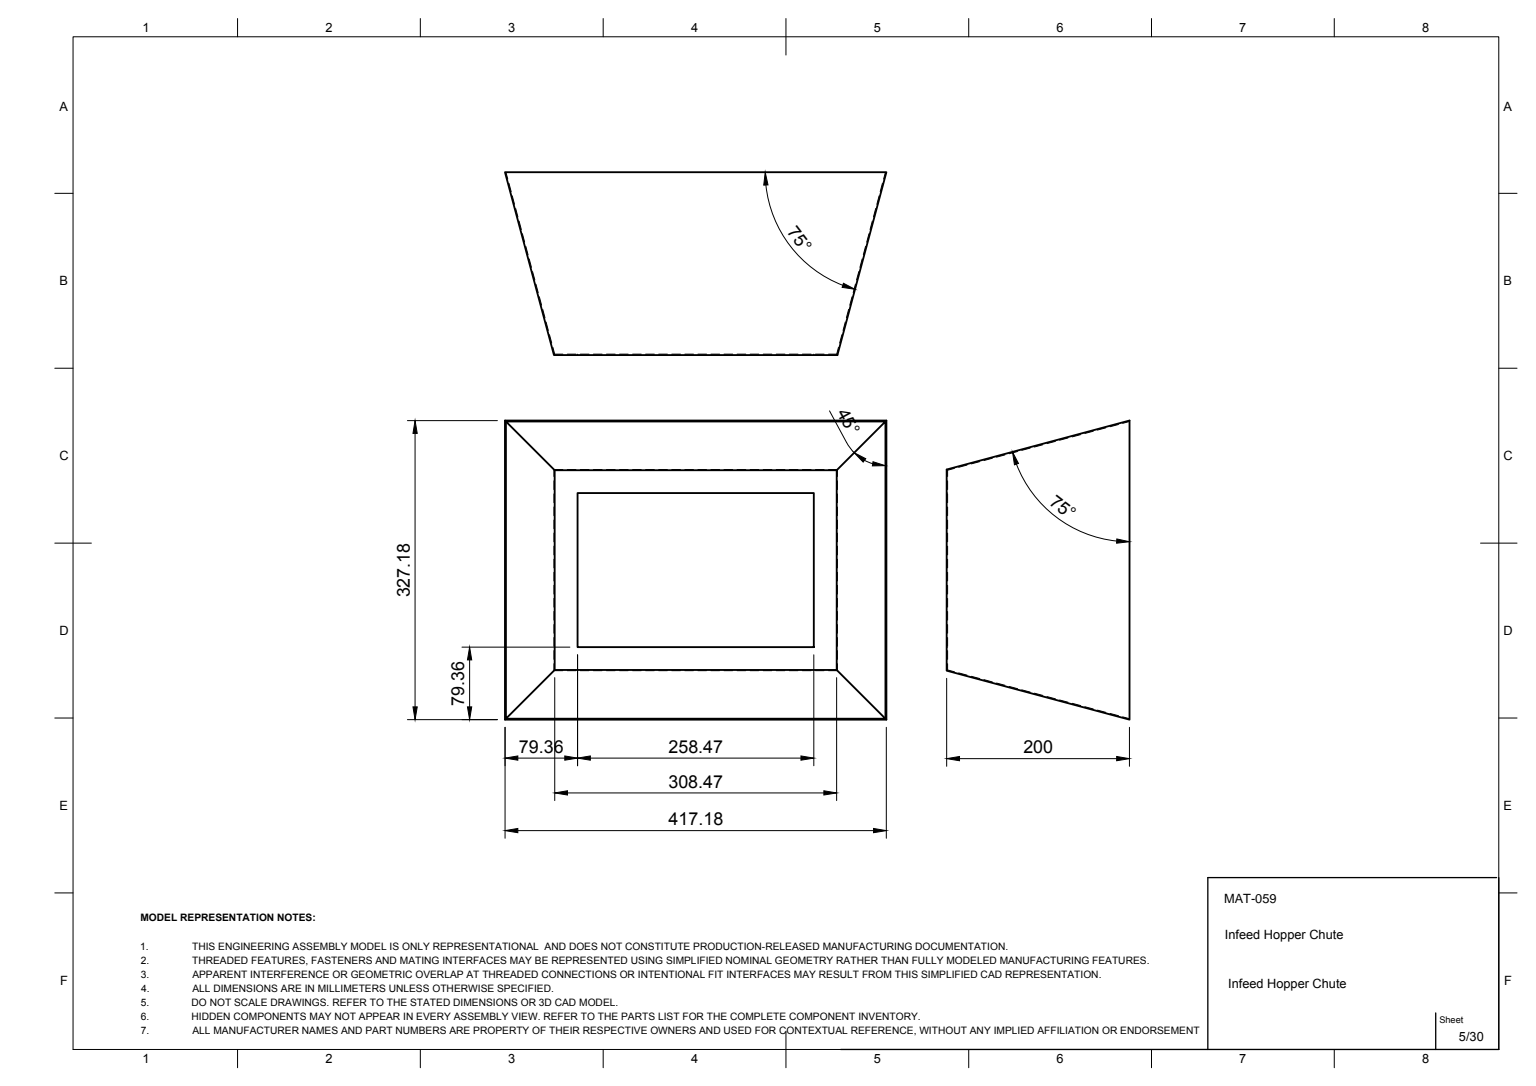
ISO-10303-21;
HEADER;
/* Generated by software containing ST-Developer
 * from STEP Tools, Inc. (www.steptools.com) 
 */

FILE_DESCRIPTION(
/* description */ ('', 'CAx-IF Rec.Pracs.---Representation and Presentation of Product Manufa
cturing Information (PMI)---4.0---2014-10-13'),
/* implementation_level */ '2;1');

FILE_NAME(
/* name */ 'Infeed Hopper Chute.step',
/* time_stamp */ '2026-10-28T23:00:48+01:00',
/* author */ (''),
/* organization */ (''),
/* preprocessor_version */ 'ST-DEVELOPER v20.2',
/* originating_system */ 'Autodesk Translation Framework v15.17.0.0',
/* authorisation */ '');

FILE_SCHEMA (('AP242_MANAGED_MODEL_BASED_3D_ENGINEERING_MIM_LF { 1 0 10303 442 2 1 4 }'));
ENDSEC;

DATA;
#10=MECHANICAL_DESIGN_GEOMETRIC_PRESENTATION_REPRESENTATION('',(#967),#61811);
#917=SHAPE_REPRESENTATION_RELATIONSHIP('SRR','None',#61975,#942);
#942=ADVANCED_BREP_SHAPE_REPRESENTATION('',(#1006),#61788);
#967=STYLED_ITEM('',(#62142),#1006);
#1006=MANIFOLD_SOLID_BREP('Body1',#33797);
#1905=FACE_BOUND('',#6351,.T.);
#1906=FACE_BOUND('',#6357,.T.);
#1907=FACE_BOUND('',#6359,.T.);
#4437=FACE_OUTER_BOUND('',#6342,.T.);
#4438=FACE_OUTER_BOUND('',#6343,.T.);
#4439=FACE_OUTER_BOUND('',#6344,.T.);
#4440=FACE_OUTER_BOUND('',#6345,.T.);
#4441=FACE_OUTER_BOUND('',#6346,.T.);
#4442=FACE_OUTER_BOUND('',#6347,.T.);
#4443=FACE_OUTER_BOUND('',#6348,.T.);
#4444=FACE_OUTER_BOUND('',#6349,.T.);
#4445=FACE_OUTER_BOUND('',#6350,.T.);
#4446=FACE_OUTER_BOUND('',#6352,.T.);
#4447=FACE_OUTER_BOUND('',#6353,.T.);
#4448=FACE_OUTER_BOUND('',#6354,.T.);
#4449=FACE_OUTER_BOUND('',#6355,.T.);
#4450=FACE_OUTER_BOUND('',#6356,.T.);
#4451=FACE_OUTER_BOUND('',#6358,.T.);
#6342=EDGE_LOOP('',(#22382,#22383,#22384,#22385));
#6343=EDGE_LOOP('',(#22386,#22387,#22388,#22389));
#6344=EDGE_LOOP('',(#22390,#22391,#22392,#22393));
#6345=EDGE_LOOP('',(#22394,#22395,#22396,#22397));
#6346=EDGE_LOOP('',(#22398,#22399,#22400,#22401));
#6347=EDGE_LOOP('',(#22402,#22403,#22404,#22405));
#6348=EDGE_LOOP('',(#22406,#22407,#22408,#22409));
#6349=EDGE_LOOP('',(#22410,#22411,#22412,#22413));
#6350=EDGE_LOOP('',(#22414,#22415,#22416,#22417));
#6351=EDGE_LOOP('',(#22418,#22419,#22420,#22421));
#6352=EDGE_LOOP('',(#22422,#22423,#22424,#22425));
#6353=EDGE_LOOP('',(#22426,#22427,#22428,#22429));
#6354=EDGE_LOOP('',(#22430,#22431,#22432,#22433));
#6355=EDGE_LOOP('',(#22434,#22435,#22436,#22437));
#6356=EDGE_LOOP('',(#22438,#22439,#22440,#22441));
#6357=EDGE_LOOP('',(#22442,#22443,#22444,#22445));
#6358=EDGE_LOOP('',(#22446,#22447,#22448,#22449));
#6359=EDGE_LOOP('',(#22450,#22451,#22452,#22453));
#8540=LINE('',#51344,#11087);
#8541=LINE('',#51346,#11088);
#8542=LINE('',#51348,#11089);
#8543=LINE('',#51349,#11090);
#8544=LINE('',#51352,#11091);
#8545=LINE('',#51354,#11092);
#8546=LINE('',#51355,#11093);
#8547=LINE('',#51358,#11094);
#8548=LINE('',#51360,#11095);
#8549=LINE('',#51361,#11096);
#8550=LINE('',#51363,#11097);
#8551=LINE('',#51364,#11098);
#8552=LINE('',#51368,#11099);
#8553=LINE('',#51370,#11100);
#8554=LINE('',#51372,#11101);
#8555=LINE('',#51373,#11102);
#8556=LINE('',#51376,#11103);
#8557=LINE('',#51378,#11104);
#8558=LINE('',#51379,#11105);
#8559=LINE('',#51382,#11106);
#8560=LINE('',#51384,#11107);
#8561=LINE('',#51385,#11108);
#8562=LINE('',#51387,#11109);
#8563=LINE('',#51388,#11110);
#8564=LINE('',#51393,#11111);
#8565=LINE('',#51395,#11112);
#8566=LINE('',#51397,#11113);
#8567=LINE('',#51398,#11114);
#8568=LINE('',#51401,#11115);
#8569=LINE('',#51403,#11116);
#8570=LINE('',#51404,#11117);
#8571=LINE('',#51407,#11118);
#8572=LINE('',#51409,#11119);
#8573=LINE('',#51410,#11120);
#8574=LINE('',#51412,#11121);
#8575=LINE('',#51413,#11122);
#11087=VECTOR('',#39164,10.);
#11088=VECTOR('',#39165,10.);
#11089=VECTOR('',#39166,10.);
#11090=VECTOR('',#39167,10.);
#11091=VECTOR('',#39170,10.);
#11092=VECTOR('',#39171,10.);
#11093=VECTOR('',#39172,10.);
#11094=VECTOR('',#39175,10.);
#11095=VECTOR('',#39176,10.);
#11096=VECTOR('',#39177,10.);
#11097=VECTOR('',#39180,10.);
#11098=VECTOR('',#39181,10.);
#11099=VECTOR('',#39184,10.);
#11100=VECTOR('',#39185,10.);
#11101=VECTOR('',#39186,10.);
#11102=VECTOR('',#39187,10.);
#11103=VECTOR('',#39190,10.);
#11104=VECTOR('',#39191,10.);
#11105=VECTOR('',#39192,10.);
#11106=VECTOR('',#39195,10.);
#11107=VECTOR('',#39196,10.);
#11108=VECTOR('',#39197,10.);
#11109=VECTOR('',#39200,10.);
#11110=VECTOR('',#39201,10.);
#11111=VECTOR('',#39206,10.);
#11112=VECTOR('',#39207,10.);
#11113=VECTOR('',#39208,10.);
#11114=VECTOR('',#39209,10.);
#11115=VECTOR('',#39212,10.);
#11116=VECTOR('',#39213,10.);
#11117=VECTOR('',#39214,10.);
#11118=VECTOR('',#39217,10.);
#11119=VECTOR('',#39218,10.);
#11120=VECTOR('',#39219,10.);
#11121=VECTOR('',#39222,10.);
#11122=VECTOR('',#39223,10.);
#13724=VERTEX_POINT('',#51342);
#13725=VERTEX_POINT('',#51343);
#13726=VERTEX_POINT('',#51345);
#13727=VERTEX_POINT('',#51347);
#13728=VERTEX_POINT('',#51351);
#13729=VERTEX_POINT('',#51353);
#13730=VERTEX_POINT('',#51357);
#13731=VERTEX_POINT('',#51359);
#13732=VERTEX_POINT('',#51366);
#13733=VERTEX_POINT('',#51367);
#13734=VERTEX_POINT('',#51369);
#13735=VERTEX_POINT('',#51371);
#13736=VERTEX_POINT('',#51375);
#13737=VERTEX_POINT('',#51377);
#13738=VERTEX_POINT('',#51381);
#13739=VERTEX_POINT('',#51383);
#13740=VERTEX_POINT('',#51391);
#13741=VERTEX_POINT('',#51392);
#13742=VERTEX_POINT('',#51394);
#13743=VERTEX_POINT('',#51396);
#13744=VERTEX_POINT('',#51400);
#13745=VERTEX_POINT('',#51402);
#13746=VERTEX_POINT('',#51406);
#13747=VERTEX_POINT('',#51408);
#17093=EDGE_CURVE('',#13724,#13725,#8540,.T.);
#17094=EDGE_CURVE('',#13726,#13724,#8541,.T.);
#17095=EDGE_CURVE('',#13727,#13726,#8542,.T.);
#17096=EDGE_CURVE('',#13727,#13725,#8543,.T.);
#17097=EDGE_CURVE('',#13725,#13728,#8544,.T.);
#17098=EDGE_CURVE('',#13729,#13727,#8545,.T.);
#17099=EDGE_CURVE('',#13729,#13728,#8546,.T.);
#17100=EDGE_CURVE('',#13728,#13730,#8547,.T.);
#17101=EDGE_CURVE('',#13731,#13729,#8548,.T.);
#17102=EDGE_CURVE('',#13731,#13730,#8549,.T.);
#17103=EDGE_CURVE('',#13730,#13724,#8550,.T.);
#17104=EDGE_CURVE('',#13726,#13731,#8551,.T.);
#17105=EDGE_CURVE('',#13732,#13733,#8552,.T.);
#17106=EDGE_CURVE('',#13734,#13732,#8553,.T.);
#17107=EDGE_CURVE('',#13735,#13734,#8554,.F.);
#17108=EDGE_CURVE('',#13735,#13733,#8555,.F.);
#17109=EDGE_CURVE('',#13733,#13736,#8556,.T.);
#17110=EDGE_CURVE('',#13737,#13735,#8557,.F.);
#17111=EDGE_CURVE('',#13737,#13736,#8558,.F.);
#17112=EDGE_CURVE('',#13736,#13738,#8559,.T.);
#17113=EDGE_CURVE('',#13739,#13737,#8560,.F.);
#17114=EDGE_CURVE('',#13739,#13738,#8561,.F.);
#17115=EDGE_CURVE('',#13738,#13732,#8562,.T.);
#17116=EDGE_CURVE('',#13734,#13739,#8563,.F.);
#17117=EDGE_CURVE('',#13740,#13741,#8564,.T.);
#17118=EDGE_CURVE('',#13742,#13741,#8565,.T.);
#17119=EDGE_CURVE('',#13742,#13743,#8566,.T.);
#17120=EDGE_CURVE('',#13743,#13740,#8567,.T.);
#17121=EDGE_CURVE('',#13741,#13744,#8568,.T.);
#17122=EDGE_CURVE('',#13745,#13744,#8569,.T.);
#17123=EDGE_CURVE('',#13745,#13742,#8570,.T.);
#17124=EDGE_CURVE('',#13744,#13746,#8571,.T.);
#17125=EDGE_CURVE('',#13747,#13746,#8572,.T.);
#17126=EDGE_CURVE('',#13747,#13745,#8573,.T.);
#17127=EDGE_CURVE('',#13746,#13740,#8574,.T.);
#17128=EDGE_CURVE('',#13743,#13747,#8575,.T.);
#22382=ORIENTED_EDGE('',*,*,#17093,.F.);
#22383=ORIENTED_EDGE('',*,*,#17094,.F.);
#22384=ORIENTED_EDGE('',*,*,#17095,.F.);
#22385=ORIENTED_EDGE('',*,*,#17096,.T.);
#22386=ORIENTED_EDGE('',*,*,#17097,.F.);
#22387=ORIENTED_EDGE('',*,*,#17096,.F.);
#22388=ORIENTED_EDGE('',*,*,#17098,.F.);
#22389=ORIENTED_EDGE('',*,*,#17099,.T.);
#22390=ORIENTED_EDGE('',*,*,#17100,.F.);
#22391=ORIENTED_EDGE('',*,*,#17099,.F.);
#22392=ORIENTED_EDGE('',*,*,#17101,.F.);
#22393=ORIENTED_EDGE('',*,*,#17102,.T.);
#22394=ORIENTED_EDGE('',*,*,#17103,.F.);
#22395=ORIENTED_EDGE('',*,*,#17102,.F.);
#22396=ORIENTED_EDGE('',*,*,#17104,.F.);
#22397=ORIENTED_EDGE('',*,*,#17094,.T.);
#22398=ORIENTED_EDGE('',*,*,#17105,.F.);
#22399=ORIENTED_EDGE('',*,*,#17106,.F.);
#22400=ORIENTED_EDGE('',*,*,#17107,.F.);
#22401=ORIENTED_EDGE('',*,*,#17108,.T.);
#22402=ORIENTED_EDGE('',*,*,#17109,.F.);
#22403=ORIENTED_EDGE('',*,*,#17108,.F.);
#22404=ORIENTED_EDGE('',*,*,#17110,.F.);
#22405=ORIENTED_EDGE('',*,*,#17111,.T.);
#22406=ORIENTED_EDGE('',*,*,#17112,.F.);
#22407=ORIENTED_EDGE('',*,*,#17111,.F.);
#22408=ORIENTED_EDGE('',*,*,#17113,.F.);
#22409=ORIENTED_EDGE('',*,*,#17114,.T.);
#22410=ORIENTED_EDGE('',*,*,#17115,.F.);
#22411=ORIENTED_EDGE('',*,*,#17114,.F.);
#22412=ORIENTED_EDGE('',*,*,#17116,.F.);
#22413=ORIENTED_EDGE('',*,*,#17106,.T.);
#22414=ORIENTED_EDGE('',*,*,#17116,.T.);
#22415=ORIENTED_EDGE('',*,*,#17113,.T.);
#22416=ORIENTED_EDGE('',*,*,#17110,.T.);
#22417=ORIENTED_EDGE('',*,*,#17107,.T.);
#22418=ORIENTED_EDGE('',*,*,#17101,.T.);
#22419=ORIENTED_EDGE('',*,*,#17098,.T.);
#22420=ORIENTED_EDGE('',*,*,#17095,.T.);
#22421=ORIENTED_EDGE('',*,*,#17104,.T.);
#22422=ORIENTED_EDGE('',*,*,#17117,.T.);
#22423=ORIENTED_EDGE('',*,*,#17118,.F.);
#22424=ORIENTED_EDGE('',*,*,#17119,.T.);
#22425=ORIENTED_EDGE('',*,*,#17120,.T.);
#22426=ORIENTED_EDGE('',*,*,#17121,.T.);
#22427=ORIENTED_EDGE('',*,*,#17122,.F.);
#22428=ORIENTED_EDGE('',*,*,#17123,.T.);
#22429=ORIENTED_EDGE('',*,*,#17118,.T.);
#22430=ORIENTED_EDGE('',*,*,#17124,.T.);
#22431=ORIENTED_EDGE('',*,*,#17125,.F.);
#22432=ORIENTED_EDGE('',*,*,#17126,.T.);
#22433=ORIENTED_EDGE('',*,*,#17122,.T.);
#22434=ORIENTED_EDGE('',*,*,#17127,.T.);
#22435=ORIENTED_EDGE('',*,*,#17120,.F.);
#22436=ORIENTED_EDGE('',*,*,#17128,.T.);
#22437=ORIENTED_EDGE('',*,*,#17125,.T.);
#22438=ORIENTED_EDGE('',*,*,#17117,.F.);
#22439=ORIENTED_EDGE('',*,*,#17127,.F.);
#22440=ORIENTED_EDGE('',*,*,#17124,.F.);
#22441=ORIENTED_EDGE('',*,*,#17121,.F.);
#22442=ORIENTED_EDGE('',*,*,#17105,.T.);
#22443=ORIENTED_EDGE('',*,*,#17109,.T.);
#22444=ORIENTED_EDGE('',*,*,#17112,.T.);
#22445=ORIENTED_EDGE('',*,*,#17115,.T.);
#22446=ORIENTED_EDGE('',*,*,#17128,.F.);
#22447=ORIENTED_EDGE('',*,*,#17119,.F.);
#22448=ORIENTED_EDGE('',*,*,#17123,.F.);
#22449=ORIENTED_EDGE('',*,*,#17126,.F.);
#22450=ORIENTED_EDGE('',*,*,#17100,.T.);
#22451=ORIENTED_EDGE('',*,*,#17103,.T.);
#22452=ORIENTED_EDGE('',*,*,#17093,.T.);
#22453=ORIENTED_EDGE('',*,*,#17097,.T.);
#31188=PLANE('',#34513);
#31189=PLANE('',#34514);
#31190=PLANE('',#34515);
#31191=PLANE('',#34516);
#31192=PLANE('',#34517);
#31193=PLANE('',#34518);
#31194=PLANE('',#34519);
#31195=PLANE('',#34520);
#31196=PLANE('',#34521);
#31197=PLANE('',#34522);
#31198=PLANE('',#34523);
#31199=PLANE('',#34524);
#31200=PLANE('',#34525);
#31201=PLANE('',#34526);
#31202=PLANE('',#34527);
#32118=ADVANCED_FACE('',(#4437),#31188,.F.);
#32119=ADVANCED_FACE('',(#4438),#31189,.F.);
#32120=ADVANCED_FACE('',(#4439),#31190,.F.);
#32121=ADVANCED_FACE('',(#4440),#31191,.F.);
#32122=ADVANCED_FACE('',(#4441),#31192,.F.);
#32123=ADVANCED_FACE('',(#4442),#31193,.F.);
#32124=ADVANCED_FACE('',(#4443),#31194,.F.);
#32125=ADVANCED_FACE('',(#4444),#31195,.F.);
#32126=ADVANCED_FACE('',(#4445,#1905),#31196,.T.);
#32127=ADVANCED_FACE('',(#4446),#31197,.T.);
#32128=ADVANCED_FACE('',(#4447),#31198,.T.);
#32129=ADVANCED_FACE('',(#4448),#31199,.T.);
#32130=ADVANCED_FACE('',(#4449),#31200,.T.);
#32131=ADVANCED_FACE('',(#4450,#1906),#31201,.T.);
#32132=ADVANCED_FACE('',(#4451,#1907),#31202,.F.);
#33797=CLOSED_SHELL('',(#32118,#32119,#32120,#32121,#32122,#32123,#32124,
#32125,#32126,#32127,#32128,#32129,#32130,#32131,#32132));
#34512=AXIS2_PLACEMENT_3D('',#51340,#39160,#39161);
#34513=AXIS2_PLACEMENT_3D('',#51341,#39162,#39163);
#34514=AXIS2_PLACEMENT_3D('',#51350,#39168,#39169);
#34515=AXIS2_PLACEMENT_3D('',#51356,#39173,#39174);
#34516=AXIS2_PLACEMENT_3D('',#51362,#39178,#39179);
#34517=AXIS2_PLACEMENT_3D('',#51365,#39182,#39183);
#34518=AXIS2_PLACEMENT_3D('',#51374,#39188,#39189);
#34519=AXIS2_PLACEMENT_3D('',#51380,#39193,#39194);
#34520=AXIS2_PLACEMENT_3D('',#51386,#39198,#39199);
#34521=AXIS2_PLACEMENT_3D('',#51389,#39202,#39203);
#34522=AXIS2_PLACEMENT_3D('',#51390,#39204,#39205);
#34523=AXIS2_PLACEMENT_3D('',#51399,#39210,#39211);
#34524=AXIS2_PLACEMENT_3D('',#51405,#39215,#39216);
#34525=AXIS2_PLACEMENT_3D('',#51411,#39220,#39221);
#34526=AXIS2_PLACEMENT_3D('',#51414,#39224,#39225);
#34527=AXIS2_PLACEMENT_3D('',#51415,#39226,#39227);
#39160=DIRECTION('axis',(0.,0.,1.));
#39161=DIRECTION('refdir',(1.,0.,0.));
#39162=DIRECTION('center_axis',(4.77727411898588E-16,1.,7.46349589431828E-16));
#39163=DIRECTION('ref_axis',(1.,-4.77727411898586E-16,-3.34404360992194E-15));
#39164=DIRECTION('',(-1.,4.77727411898586E-16,3.34404360992194E-15));
#39165=DIRECTION('',(-3.34404360992194E-15,7.4634958943183E-16,-1.));
#39166=DIRECTION('',(1.,-4.77727411898586E-16,-3.34404360992194E-15));
#39167=DIRECTION('',(-3.34404360992194E-15,7.4634958943183E-16,-1.));
#39168=DIRECTION('center_axis',(-1.,4.77727411898586E-16,3.34404360992194E-15));
#39169=DIRECTION('ref_axis',(4.77727411898588E-16,1.,7.46349589431829E-16));
#39170=DIRECTION('',(-4.77727411898588E-16,-1.,-7.46349589431828E-16));
#39171=DIRECTION('',(4.77727411898588E-16,1.,7.46349589431828E-16));
#39172=DIRECTION('',(-3.34404360992194E-15,7.4634958943183E-16,-1.));
#39173=DIRECTION('center_axis',(-4.77727411898588E-16,-1.,-7.46349589431828E-16));
#39174=DIRECTION('ref_axis',(-1.,4.77727411898586E-16,3.34404360992194E-15));
#39175=DIRECTION('',(1.,-4.77727411898586E-16,-3.34404360992194E-15));
#39176=DIRECTION('',(-1.,4.77727411898586E-16,3.34404360992194E-15));
#39177=DIRECTION('',(-3.34404360992194E-15,7.4634958943183E-16,-1.));
#39178=DIRECTION('center_axis',(1.,-4.77727411898586E-16,-3.34404360992194E-15));
#39179=DIRECTION('ref_axis',(-4.77727411898588E-16,-1.,-7.46349589431829E-16));
#39180=DIRECTION('',(4.77727411898588E-16,1.,7.46349589431828E-16));
#39181=DIRECTION('',(-4.77727411898588E-16,-1.,-7.46349589431828E-16));
#39182=DIRECTION('center_axis',(-3.81963526526752E-16,0.965925826289068,
-0.25881904510252));
#39183=DIRECTION('ref_axis',(-1.,5.00596043934458E-16,3.34404360992194E-15));
#39184=DIRECTION('',(1.,-5.00596043934458E-16,-3.34404360992194E-15));
#39185=DIRECTION('',(-0.250562807085729,0.250562807085731,0.93511312653103));
#39186=DIRECTION('',(1.,-5.00596043934458E-16,-3.34404360992194E-15));
#39187=DIRECTION('',(-0.250562807085735,-0.250562807085731,-0.935113126531028));
#39188=DIRECTION('center_axis',(0.965925826289067,-2.90369159325025E-16,
-0.258819045102524));
#39189=DIRECTION('ref_axis',(5.0059604393446E-16,1.,7.46349589431828E-16));
#39190=DIRECTION('',(-5.0059604393446E-16,-1.,-7.46349589431828E-16));
#39191=DIRECTION('',(-5.0059604393446E-16,-1.,-7.46349589431828E-16));
#39192=DIRECTION('',(-0.250562807085735,0.250562807085733,-0.935113126531028));
#39193=DIRECTION('center_axis',(-1.34904082127562E-15,-0.965925826289068,
-0.258819045102522));
#39194=DIRECTION('ref_axis',(1.,-5.00596043934458E-16,-3.34404360992194E-15));
#39195=DIRECTION('',(-1.,5.00596043934458E-16,3.34404360992194E-15));
#39196=DIRECTION('',(-1.,5.00596043934458E-16,3.34404360992194E-15));
#39197=DIRECTION('',(0.250562807085729,0.250562807085733,-0.93511312653103));
#39198=DIRECTION('center_axis',(-0.965925826289069,6.76708135423834E-16,
-0.258819045102518));
#39199=DIRECTION('ref_axis',(-5.0059604393446E-16,-1.,-7.46349589431828E-16));
#39200=DIRECTION('',(5.0059604393446E-16,1.,7.46349589431828E-16));
#39201=DIRECTION('',(5.0059604393446E-16,1.,7.46349589431828E-16));
#39202=DIRECTION('center_axis',(3.34404360992194E-15,-7.4634958943183E-16,
1.));
#39203=DIRECTION('ref_axis',(-5.0059604393446E-16,-1.,-7.46349589431828E-16));
#39204=DIRECTION('center_axis',(-3.81963526526752E-16,0.965925826289068,
-0.25881904510252));
#39205=DIRECTION('ref_axis',(-1.,5.00596043934458E-16,3.34404360992194E-15));
#39206=DIRECTION('',(1.,-5.00596043934458E-16,-3.34404360992194E-15));
#39207=DIRECTION('',(0.250562807085735,0.250562807085731,0.935113126531028));
#39208=DIRECTION('',(-1.,5.00596043934458E-16,3.34404360992194E-15));
#39209=DIRECTION('',(-0.250562807085729,0.250562807085731,0.93511312653103));
#39210=DIRECTION('center_axis',(0.965925826289067,-2.90369159325025E-16,
-0.258819045102524));
#39211=DIRECTION('ref_axis',(5.0059604393446E-16,1.,7.46349589431828E-16));
#39212=DIRECTION('',(-5.0059604393446E-16,-1.,-7.46349589431828E-16));
#39213=DIRECTION('',(0.250562807085735,-0.250562807085733,0.935113126531028));
#39214=DIRECTION('',(5.0059604393446E-16,1.,7.46349589431828E-16));
#39215=DIRECTION('center_axis',(-1.34904082127562E-15,-0.965925826289068,
-0.258819045102522));
#39216=DIRECTION('ref_axis',(1.,-5.00596043934458E-16,-3.34404360992194E-15));
#39217=DIRECTION('',(-1.,5.00596043934458E-16,3.34404360992194E-15));
#39218=DIRECTION('',(-0.250562807085729,-0.250562807085733,0.93511312653103));
#39219=DIRECTION('',(1.,-5.00596043934458E-16,-3.34404360992194E-15));
#39220=DIRECTION('center_axis',(-0.965925826289069,6.76708135423834E-16,
-0.258819045102518));
#39221=DIRECTION('ref_axis',(-5.0059604393446E-16,-1.,-7.46349589431828E-16));
#39222=DIRECTION('',(5.0059604393446E-16,1.,7.46349589431828E-16));
#39223=DIRECTION('',(-5.0059604393446E-16,-1.,-7.46349589431828E-16));
#39224=DIRECTION('center_axis',(3.34404360992194E-15,-7.4634958943183E-16,
1.));
#39225=DIRECTION('ref_axis',(-5.0059604393446E-16,-1.,-7.46349589431828E-16));
#39226=DIRECTION('center_axis',(3.34404360992194E-15,-7.4634958943183E-16,
1.));
#39227=DIRECTION('ref_axis',(-5.0059604393446E-16,-1.,-7.46349589431828E-16));
#51340=CARTESIAN_POINT('',(0.,0.,0.));
#51341=CARTESIAN_POINT('Origin',(189.88324475895,-96.2393342567687,531.000000551894));
#51342=CARTESIAN_POINT('',(448.348590782989,-96.2393342567688,530.000000551893));
#51343=CARTESIAN_POINT('',(189.88324475895,-96.2393342567687,530.000000551894));
#51344=CARTESIAN_POINT('',(254.49958126496,-96.2393342567687,530.000000551894));
#51345=CARTESIAN_POINT('',(448.348590782989,-96.2393342567688,531.000000551893));
#51346=CARTESIAN_POINT('',(448.348590782989,-96.2393342567688,531.000000551893));
#51347=CARTESIAN_POINT('',(189.88324475895,-96.2393342567687,531.000000551894));
#51348=CARTESIAN_POINT('',(254.49958126496,-96.2393342567687,531.000000551894));
#51349=CARTESIAN_POINT('',(189.88324475895,-96.2393342567687,531.000000551894));
#51350=CARTESIAN_POINT('Origin',(189.88324475895,-264.704680280811,531.000000551894));
#51351=CARTESIAN_POINT('',(189.88324475895,-264.704680280811,530.000000551894));
#51352=CARTESIAN_POINT('',(189.88324475895,-222.5883437748,530.000000551894));
#51353=CARTESIAN_POINT('',(189.88324475895,-264.704680280811,531.000000551894));
#51354=CARTESIAN_POINT('',(189.88324475895,-222.5883437748,531.000000551894));
#51355=CARTESIAN_POINT('',(189.88324475895,-264.704680280811,531.000000551894));
#51356=CARTESIAN_POINT('Origin',(448.348590782989,-264.704680280811,531.000000551893));
#51357=CARTESIAN_POINT('',(448.348590782989,-264.704680280811,530.000000551893));
#51358=CARTESIAN_POINT('',(383.73225427698,-264.704680280811,530.000000551893));
#51359=CARTESIAN_POINT('',(448.348590782989,-264.704680280811,531.000000551893));
#51360=CARTESIAN_POINT('',(383.73225427698,-264.704680280811,531.000000551893));
#51361=CARTESIAN_POINT('',(448.348590782989,-264.704680280811,531.000000551893));
#51362=CARTESIAN_POINT('Origin',(448.348590782989,-96.2393342567688,531.000000551893));
#51363=CARTESIAN_POINT('',(448.348590782989,-138.355670762779,530.000000551893));
#51364=CARTESIAN_POINT('',(448.348590782989,-138.355670762779,531.000000551893));
#51365=CARTESIAN_POINT('Origin',(164.115917770971,-71.4379330950788,530.258819596997));
#51366=CARTESIAN_POINT('',(111.561355465157,-17.9174449629754,730.000000551894));
#51367=CARTESIAN_POINT('',(526.670480076784,-17.9174449629756,730.000000551893));
#51368=CARTESIAN_POINT('',(241.615917770971,-17.9174449629754,730.000000551894));
#51369=CARTESIAN_POINT('',(164.88324475895,-71.2393342567687,531.000000551894));
#51370=CARTESIAN_POINT('',(171.927190344623,-78.2832798424422,504.71163774041));
#51371=CARTESIAN_POINT('',(473.348590782989,-71.2393342567688,531.000000551893));
#51372=CARTESIAN_POINT('',(241.61591777097,-71.2393342567687,531.000000551894));
#51373=CARTESIAN_POINT('',(463.479467784055,-81.1084572557029,494.167932093724));
#51374=CARTESIAN_POINT('Origin',(473.149991944679,-70.4720072687899,530.258819596996));
#51375=CARTESIAN_POINT('',(526.670480076784,-343.026569574604,730.000000551893));
#51376=CARTESIAN_POINT('',(526.670480076784,-125.47200726879,730.000000551893));
#51377=CARTESIAN_POINT('',(473.348590782989,-289.704680280811,531.000000551893));
#51378=CARTESIAN_POINT('',(473.348590782989,-125.47200726879,531.000000551893));
#51379=CARTESIAN_POINT('',(466.304645197316,-282.660734695137,504.711637740409));
#51380=CARTESIAN_POINT('Origin',(474.115917770968,-289.506081442501,530.258819596995));
#51381=CARTESIAN_POINT('',(111.561355465157,-343.026569574604,730.000000551894));
#51382=CARTESIAN_POINT('',(396.61591777097,-343.026569574604,730.000000551893));
#51383=CARTESIAN_POINT('',(164.88324475895,-289.704680280811,531.000000551894));
#51384=CARTESIAN_POINT('',(396.615917770969,-289.704680280811,531.000000551893));
#51385=CARTESIAN_POINT('',(174.752367757884,-279.835557281876,494.167932093725));
#51386=CARTESIAN_POINT('Origin',(165.08184359726,-290.47200726879,530.258819596996));
#51387=CARTESIAN_POINT('',(111.561355465157,-235.47200726879,730.000000551894));
#51388=CARTESIAN_POINT('',(164.88324475895,-235.47200726879,531.000000551894));
#51389=CARTESIAN_POINT('Origin',(319.11591777097,-180.47200726879,531.000000551893));
#51390=CARTESIAN_POINT('Origin',(164.115917770971,-70.4720072687897,530.000000551894));
#51391=CARTESIAN_POINT('',(110.526079284747,-16.8821687825653,730.000000551894));
#51392=CARTESIAN_POINT('',(527.705756257194,-16.8821687825655,730.000000551893));
#51393=CARTESIAN_POINT('',(474.115917770969,-16.8821687825655,730.000000551893));
#51394=CARTESIAN_POINT('',(474.115917770968,-70.4720072687899,530.000000551893));
#51395=CARTESIAN_POINT('',(464.384751125293,-80.2031739144654,493.682792213312));
#51396=CARTESIAN_POINT('',(164.115917770971,-70.4720072687897,530.000000551894));
#51397=CARTESIAN_POINT('',(474.115917770968,-70.4720072687899,530.000000551893));
#51398=CARTESIAN_POINT('',(171.021907003386,-77.3779965012046,504.226497859998));
#51399=CARTESIAN_POINT('Origin',(474.115917770968,-70.4720072687899,530.000000551893));
#51400=CARTESIAN_POINT('',(527.705756257194,-344.061845755014,730.000000551893));
#51401=CARTESIAN_POINT('',(527.705756257194,-290.47200726879,730.000000551893));
#51402=CARTESIAN_POINT('',(474.115917770968,-290.47200726879,530.000000551893));
#51403=CARTESIAN_POINT('',(467.209928538553,-283.566018036375,504.226497859997));
#51404=CARTESIAN_POINT('',(474.115917770968,-290.47200726879,530.000000551893));
#51405=CARTESIAN_POINT('Origin',(474.115917770968,-290.47200726879,530.000000551893));
#51406=CARTESIAN_POINT('',(110.526079284747,-344.061845755014,730.000000551894));
#51407=CARTESIAN_POINT('',(164.115917770972,-344.061845755014,730.000000551894));
#51408=CARTESIAN_POINT('',(164.115917770971,-290.47200726879,530.000000551894));
#51409=CARTESIAN_POINT('',(173.847084416646,-280.740840623114,493.682792213313));
#51410=CARTESIAN_POINT('',(164.115917770971,-290.47200726879,530.000000551894));
#51411=CARTESIAN_POINT('Origin',(164.115917770971,-290.47200726879,530.000000551894));
#51412=CARTESIAN_POINT('',(110.526079284747,-70.4720072687898,730.000000551894));
#51413=CARTESIAN_POINT('',(164.115917770971,-70.4720072687897,530.000000551894));
#51414=CARTESIAN_POINT('Origin',(319.115917770971,-180.47200726879,730.000000551893));
#51415=CARTESIAN_POINT('Origin',(319.11591777097,-180.47200726879,530.000000551893));
#61757=UNCERTAINTY_MEASURE_WITH_UNIT(LENGTH_MEASURE(0.01),#61812,
'DISTANCE_ACCURACY_VALUE',
'Maximum model space distance between geometric entities at asserted c
onnectivities');
#61780=UNCERTAINTY_MEASURE_WITH_UNIT(LENGTH_MEASURE(0.01),#61812,
'DISTANCE_ACCURACY_VALUE',
'Maximum model space distance between geometric entities at asserted c
onnectivities');
#61788=(
GEOMETRIC_REPRESENTATION_CONTEXT(3)
GLOBAL_UNCERTAINTY_ASSIGNED_CONTEXT((#61757))
GLOBAL_UNIT_ASSIGNED_CONTEXT((#61812,#61814,#61815))
REPRESENTATION_CONTEXT('','3D')
);
#61811=(
GEOMETRIC_REPRESENTATION_CONTEXT(3)
GLOBAL_UNCERTAINTY_ASSIGNED_CONTEXT((#61780))
GLOBAL_UNIT_ASSIGNED_CONTEXT((#61812,#61814,#61815))
REPRESENTATION_CONTEXT('','3D')
);
#61812=(
LENGTH_UNIT()
NAMED_UNIT(*)
SI_UNIT(.MILLI.,.METRE.)
);
#61814=(
NAMED_UNIT(*)
PLANE_ANGLE_UNIT()
SI_UNIT($,.RADIAN.)
);
#61815=(
NAMED_UNIT(*)
SI_UNIT($,.STERADIAN.)
SOLID_ANGLE_UNIT()
);
#61823=SHAPE_DEFINITION_REPRESENTATION(#61853,#61975);
#61853=PRODUCT_DEFINITION_SHAPE('',$,#62006);
#61975=SHAPE_REPRESENTATION('',(#34512),#61788);
#61998=PRODUCT_DEFINITION_CONTEXT('part definition',#62090,'design');
#62006=PRODUCT_DEFINITION('Infeed Hopper Chute','Infeed Hopper Chute',#62036,
#61998);
#62036=PRODUCT_DEFINITION_FORMATION('',$,#62099);
#62090=APPLICATION_CONTEXT('Managed model based 3d engineering');
#62091=PRODUCT_CONTEXT('part definition',#62090,'mechanical');
#62099=PRODUCT('Infeed Hopper Chute','Infeed Hopper Chute',$,(#62091));
#62136=COLOUR_RGB('Light Blue',0.38,0.62,0.78);
#62137=FILL_AREA_STYLE_COLOUR('',#62136);
#62138=FILL_AREA_STYLE('',(#62137));
#62139=SURFACE_STYLE_FILL_AREA(#62138);
#62140=SURFACE_SIDE_STYLE('',(#62139));
#62141=SURFACE_STYLE_USAGE(.BOTH.,#62140);
#62142=PRESENTATION_STYLE_ASSIGNMENT((#62141));
ENDSEC;
END-ISO-10303-21;
